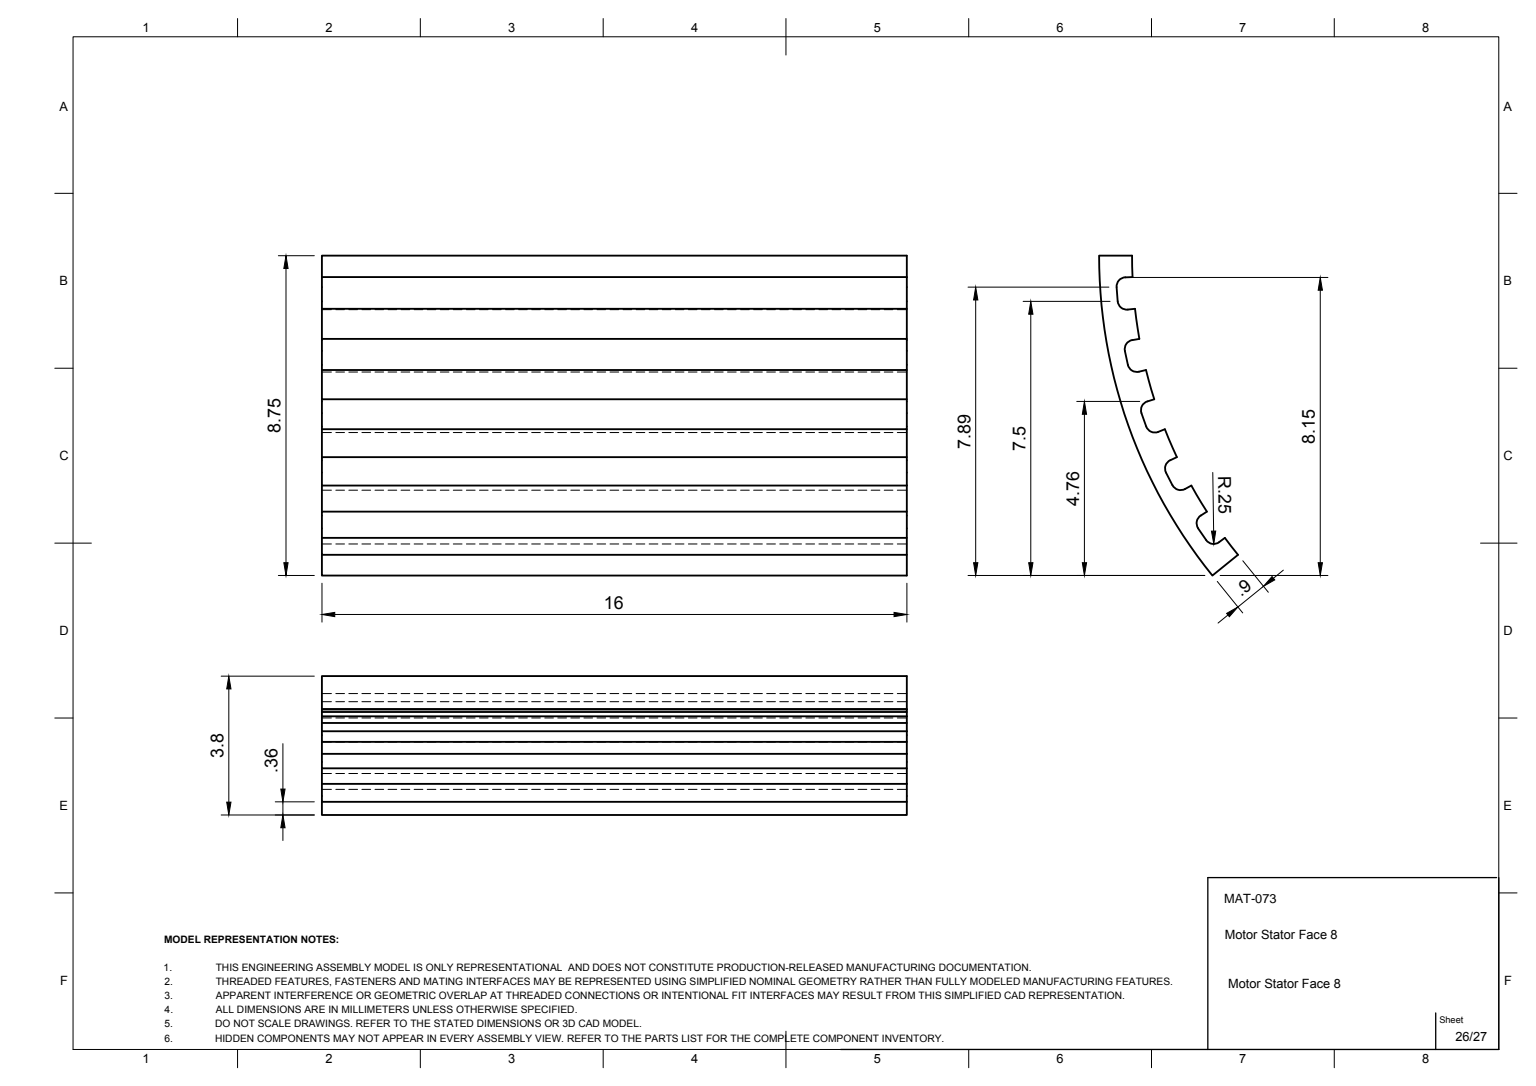
ISO-10303-21;
HEADER;
/* Generated by software containing ST-Developer
 * from STEP Tools, Inc. (www.steptools.com) 
 */

FILE_DESCRIPTION(
/* description */ ('CAx-IF Rec.Pracs.---Representation and Presentation of Product Manufa
cturing Information (PMI)---4.0---2014-10-13'),
/* implementation_level */ '2;1');

FILE_NAME(
/* name */ 'Motor Stator Face 8.step',
/* time_stamp */ '2026-10-24T18:52:33-07:00',
/* author */ (''),
/* organization */ (''),
/* preprocessor_version */ 'ST-DEVELOPER v20.2',
/* originating_system */ 'Autodesk Translation Framework v15.17.0.0',
/* authorisation */ '');

FILE_SCHEMA (('AP242_MANAGED_MODEL_BASED_3D_ENGINEERING_MIM_LF { 1 0 10303 442 2 1 4 }'));
ENDSEC;

DATA;
#10=MECHANICAL_DESIGN_GEOMETRIC_PRESENTATION_REPRESENTATION('',(#443),#34876);
#377=SHAPE_REPRESENTATION_RELATIONSHIP('SRR','None',#35014,#410);
#410=ADVANCED_BREP_SHAPE_REPRESENTATION('',(#476),#34872);
#443=STYLED_ITEM('',(#35163),#476);
#476=MANIFOLD_SOLID_BREP('Motor Stator Face 8',#19583);
#1049=PLANE('',#22059);
#1050=PLANE('',#22069);
#1051=PLANE('',#22079);
#1052=PLANE('',#22089);
#1053=PLANE('',#22099);
#1054=PLANE('',#22100);
#1055=PLANE('',#22101);
#1056=PLANE('',#22102);
#1057=PLANE('',#22103);
#1058=PLANE('',#22110);
#1059=PLANE('',#22120);
#1060=PLANE('',#22123);
#1061=PLANE('',#22126);
#1062=PLANE('',#22129);
#2589=LINE('',#34145,#4188);
#2590=LINE('',#34148,#4189);
#2591=LINE('',#34153,#4190);
#2592=LINE('',#34159,#4191);
#2593=LINE('',#34163,#4192);
#2594=LINE('',#34165,#4193);
#2595=LINE('',#34166,#4194);
#2596=LINE('',#34172,#4195);
#2597=LINE('',#34175,#4196);
#2598=LINE('',#34180,#4197);
#2599=LINE('',#34186,#4198);
#2600=LINE('',#34190,#4199);
#2601=LINE('',#34192,#4200);
#2602=LINE('',#34193,#4201);
#2603=LINE('',#34199,#4202);
#2604=LINE('',#34202,#4203);
#2605=LINE('',#34207,#4204);
#2606=LINE('',#34213,#4205);
#2607=LINE('',#34217,#4206);
#2608=LINE('',#34219,#4207);
#2609=LINE('',#34220,#4208);
#2610=LINE('',#34226,#4209);
#2611=LINE('',#34229,#4210);
#2612=LINE('',#34234,#4211);
#2613=LINE('',#34240,#4212);
#2614=LINE('',#34244,#4213);
#2615=LINE('',#34246,#4214);
#2616=LINE('',#34247,#4215);
#2617=LINE('',#34253,#4216);
#2618=LINE('',#34256,#4217);
#2619=LINE('',#34261,#4218);
#2620=LINE('',#34267,#4219);
#2621=LINE('',#34271,#4220);
#2622=LINE('',#34273,#4221);
#2623=LINE('',#34274,#4222);
#2624=LINE('',#34277,#4223);
#2625=LINE('',#34279,#4224);
#2626=LINE('',#34280,#4225);
#2627=LINE('',#34283,#4226);
#2628=LINE('',#34285,#4227);
#2629=LINE('',#34286,#4228);
#2630=LINE('',#34289,#4229);
#2631=LINE('',#34291,#4230);
#2632=LINE('',#34292,#4231);
#2633=LINE('',#34295,#4232);
#2634=LINE('',#34297,#4233);
#2635=LINE('',#34298,#4234);
#2636=LINE('',#34303,#4235);
#2637=LINE('',#34310,#4236);
#2638=LINE('',#34314,#4237);
#2639=LINE('',#34319,#4238);
#2640=LINE('',#34324,#4239);
#2641=LINE('',#34327,#4240);
#2642=LINE('',#34330,#4241);
#2643=LINE('',#34335,#4242);
#2644=LINE('',#34336,#4243);
#2645=LINE('',#34340,#4244);
#2646=LINE('',#34342,#4245);
#4188=VECTOR('',#27966,1.);
#4189=VECTOR('',#27969,1.);
#4190=VECTOR('',#27974,1.);
#4191=VECTOR('',#27981,1.);
#4192=VECTOR('',#27986,1.);
#4193=VECTOR('',#27987,1.);
#4194=VECTOR('',#27988,1.);
#4195=VECTOR('',#27993,1.);
#4196=VECTOR('',#27996,1.);
#4197=VECTOR('',#28001,1.);
#4198=VECTOR('',#28008,1.);
#4199=VECTOR('',#28013,0.999999999999999);
#4200=VECTOR('',#28014,1.);
#4201=VECTOR('',#28015,0.999999999999999);
#4202=VECTOR('',#28020,1.);
#4203=VECTOR('',#28023,1.);
#4204=VECTOR('',#28028,1.);
#4205=VECTOR('',#28035,1.);
#4206=VECTOR('',#28040,1.);
#4207=VECTOR('',#28041,1.);
#4208=VECTOR('',#28042,1.);
#4209=VECTOR('',#28047,1.);
#4210=VECTOR('',#28050,1.);
#4211=VECTOR('',#28055,1.);
#4212=VECTOR('',#28062,1.);
#4213=VECTOR('',#28067,1.);
#4214=VECTOR('',#28068,1.);
#4215=VECTOR('',#28069,1.);
#4216=VECTOR('',#28074,1.);
#4217=VECTOR('',#28077,1.);
#4218=VECTOR('',#28082,1.);
#4219=VECTOR('',#28089,1.);
#4220=VECTOR('',#28094,1.);
#4221=VECTOR('',#28095,1.);
#4222=VECTOR('',#28096,1.);
#4223=VECTOR('',#28099,1.);
#4224=VECTOR('',#28100,1.);
#4225=VECTOR('',#28101,1.);
#4226=VECTOR('',#28104,0.999999999999999);
#4227=VECTOR('',#28105,1.);
#4228=VECTOR('',#28106,0.999999999999999);
#4229=VECTOR('',#28109,1.);
#4230=VECTOR('',#28110,1.);
#4231=VECTOR('',#28111,1.);
#4232=VECTOR('',#28114,1.);
#4233=VECTOR('',#28115,1.);
#4234=VECTOR('',#28116,1.);
#4235=VECTOR('',#28121,1.);
#4236=VECTOR('',#28132,1.);
#4237=VECTOR('',#28135,1.);
#4238=VECTOR('',#28142,1.);
#4239=VECTOR('',#28149,1.);
#4240=VECTOR('',#28152,1.);
#4241=VECTOR('',#28157,1.);
#4242=VECTOR('',#28164,1.);
#4243=VECTOR('',#28165,1.);
#4244=VECTOR('',#28170,1.);
#4245=VECTOR('',#28173,1.);
#4766=CYLINDRICAL_SURFACE('',#22050,0.00025);
#4767=CYLINDRICAL_SURFACE('',#22053,0.01345);
#4768=CYLINDRICAL_SURFACE('',#22056,0.00025);
#4769=CYLINDRICAL_SURFACE('',#22060,0.00025);
#4770=CYLINDRICAL_SURFACE('',#22063,0.01345);
#4771=CYLINDRICAL_SURFACE('',#22066,0.00025);
#4772=CYLINDRICAL_SURFACE('',#22070,0.00025);
#4773=CYLINDRICAL_SURFACE('',#22073,0.01345);
#4774=CYLINDRICAL_SURFACE('',#22076,0.00025);
#4775=CYLINDRICAL_SURFACE('',#22080,0.00025);
#4776=CYLINDRICAL_SURFACE('',#22083,0.01345);
#4777=CYLINDRICAL_SURFACE('',#22086,0.00025);
#4778=CYLINDRICAL_SURFACE('',#22090,0.00025);
#4779=CYLINDRICAL_SURFACE('',#22093,0.01345);
#4780=CYLINDRICAL_SURFACE('',#22096,0.00025);
#4781=CYLINDRICAL_SURFACE('',#22104,0.013);
#4782=CYLINDRICAL_SURFACE('',#22107,0.013);
#4783=CYLINDRICAL_SURFACE('',#22116,0.013);
#4784=CYLINDRICAL_SURFACE('',#22118,0.013);
#4785=CYLINDRICAL_SURFACE('',#22121,0.013);
#4786=CYLINDRICAL_SURFACE('',#22124,0.0139);
#4787=CYLINDRICAL_SURFACE('',#22127,0.013);
#5757=FACE_OUTER_BOUND('',#6908,.T.);
#5758=FACE_OUTER_BOUND('',#6909,.T.);
#5759=FACE_OUTER_BOUND('',#6910,.T.);
#5760=FACE_OUTER_BOUND('',#6911,.T.);
#5761=FACE_OUTER_BOUND('',#6912,.T.);
#5762=FACE_OUTER_BOUND('',#6913,.T.);
#5763=FACE_OUTER_BOUND('',#6914,.T.);
#5764=FACE_OUTER_BOUND('',#6915,.T.);
#5765=FACE_OUTER_BOUND('',#6916,.T.);
#5766=FACE_OUTER_BOUND('',#6917,.T.);
#5767=FACE_OUTER_BOUND('',#6918,.T.);
#5768=FACE_OUTER_BOUND('',#6919,.T.);
#5769=FACE_OUTER_BOUND('',#6920,.T.);
#5770=FACE_OUTER_BOUND('',#6921,.T.);
#5771=FACE_OUTER_BOUND('',#6922,.T.);
#5772=FACE_OUTER_BOUND('',#6923,.T.);
#5773=FACE_OUTER_BOUND('',#6924,.T.);
#5774=FACE_OUTER_BOUND('',#6925,.T.);
#5775=FACE_OUTER_BOUND('',#6926,.T.);
#5776=FACE_OUTER_BOUND('',#6927,.T.);
#5777=FACE_OUTER_BOUND('',#6928,.T.);
#5778=FACE_OUTER_BOUND('',#6929,.T.);
#5779=FACE_OUTER_BOUND('',#6930,.T.);
#5780=FACE_OUTER_BOUND('',#6931,.T.);
#5781=FACE_OUTER_BOUND('',#6932,.T.);
#5782=FACE_OUTER_BOUND('',#6933,.T.);
#5783=FACE_OUTER_BOUND('',#6934,.T.);
#5784=FACE_OUTER_BOUND('',#6935,.T.);
#5785=FACE_OUTER_BOUND('',#6936,.T.);
#5786=FACE_OUTER_BOUND('',#6937,.T.);
#5787=FACE_OUTER_BOUND('',#6938,.T.);
#5788=FACE_OUTER_BOUND('',#6939,.T.);
#5789=FACE_OUTER_BOUND('',#6940,.T.);
#5790=FACE_OUTER_BOUND('',#6941,.T.);
#5791=FACE_OUTER_BOUND('',#6942,.T.);
#5792=FACE_OUTER_BOUND('',#6943,.T.);
#6908=EDGE_LOOP('',(#18070,#18071,#18072,#18073));
#6909=EDGE_LOOP('',(#18074,#18075,#18076,#18077));
#6910=EDGE_LOOP('',(#18078,#18079,#18080,#18081));
#6911=EDGE_LOOP('',(#18082,#18083,#18084,#18085));
#6912=EDGE_LOOP('',(#18086,#18087,#18088,#18089));
#6913=EDGE_LOOP('',(#18090,#18091,#18092,#18093));
#6914=EDGE_LOOP('',(#18094,#18095,#18096,#18097));
#6915=EDGE_LOOP('',(#18098,#18099,#18100,#18101));
#6916=EDGE_LOOP('',(#18102,#18103,#18104,#18105));
#6917=EDGE_LOOP('',(#18106,#18107,#18108,#18109));
#6918=EDGE_LOOP('',(#18110,#18111,#18112,#18113));
#6919=EDGE_LOOP('',(#18114,#18115,#18116,#18117));
#6920=EDGE_LOOP('',(#18118,#18119,#18120,#18121));
#6921=EDGE_LOOP('',(#18122,#18123,#18124,#18125));
#6922=EDGE_LOOP('',(#18126,#18127,#18128,#18129));
#6923=EDGE_LOOP('',(#18130,#18131,#18132,#18133));
#6924=EDGE_LOOP('',(#18134,#18135,#18136,#18137));
#6925=EDGE_LOOP('',(#18138,#18139,#18140,#18141));
#6926=EDGE_LOOP('',(#18142,#18143,#18144,#18145));
#6927=EDGE_LOOP('',(#18146,#18147,#18148,#18149));
#6928=EDGE_LOOP('',(#18150,#18151,#18152,#18153));
#6929=EDGE_LOOP('',(#18154,#18155,#18156,#18157));
#6930=EDGE_LOOP('',(#18158,#18159,#18160,#18161));
#6931=EDGE_LOOP('',(#18162,#18163,#18164,#18165));
#6932=EDGE_LOOP('',(#18166,#18167,#18168,#18169));
#6933=EDGE_LOOP('',(#18170,#18171,#18172,#18173));
#6934=EDGE_LOOP('',(#18174,#18175,#18176,#18177,#18178,#18179,#18180,#18181,
#18182,#18183,#18184,#18185,#18186,#18187,#18188,#18189,#18190,#18191,#18192,
#18193,#18194,#18195,#18196,#18197,#18198,#18199,#18200,#18201,#18202,#18203,
#18204,#18205,#18206,#18207));
#6935=EDGE_LOOP('',(#18208,#18209,#18210,#18211));
#6936=EDGE_LOOP('',(#18212,#18213,#18214,#18215));
#6937=EDGE_LOOP('',(#18216,#18217,#18218,#18219));
#6938=EDGE_LOOP('',(#18220,#18221,#18222,#18223));
#6939=EDGE_LOOP('',(#18224,#18225,#18226,#18227));
#6940=EDGE_LOOP('',(#18228,#18229,#18230,#18231));
#6941=EDGE_LOOP('',(#18232,#18233,#18234,#18235));
#6942=EDGE_LOOP('',(#18236,#18237,#18238,#18239));
#6943=EDGE_LOOP('',(#18240,#18241,#18242,#18243,#18244,#18245,#18246,#18247,
#18248,#18249,#18250,#18251,#18252,#18253,#18254,#18255,#18256,#18257,#18258,
#18259,#18260,#18261,#18262,#18263,#18264,#18265,#18266,#18267,#18268,#18269,
#18270,#18271,#18272,#18273));
#7985=CIRCLE('',#22051,0.000250000000012414);
#7986=CIRCLE('',#22052,0.000250000000012414);
#7987=CIRCLE('',#22054,0.0134500000000135);
#7988=CIRCLE('',#22055,0.0134500000000135);
#7989=CIRCLE('',#22057,0.000250000000012074);
#7990=CIRCLE('',#22058,0.000250000000012074);
#7991=CIRCLE('',#22061,0.000250000000011423);
#7992=CIRCLE('',#22062,0.000250000000011423);
#7993=CIRCLE('',#22064,0.0134500000000139);
#7994=CIRCLE('',#22065,0.0134500000000139);
#7995=CIRCLE('',#22067,0.00025000000001101);
#7996=CIRCLE('',#22068,0.00025000000001101);
#7997=CIRCLE('',#22071,0.000250000000010237);
#7998=CIRCLE('',#22072,0.000250000000010237);
#7999=CIRCLE('',#22074,0.0134500000000141);
#8000=CIRCLE('',#22075,0.0134500000000141);
#8001=CIRCLE('',#22077,0.000250000000010237);
#8002=CIRCLE('',#22078,0.000250000000010237);
#8003=CIRCLE('',#22081,0.00025000000001101);
#8004=CIRCLE('',#22082,0.00025000000001101);
#8005=CIRCLE('',#22084,0.0134500000000141);
#8006=CIRCLE('',#22085,0.0134500000000141);
#8007=CIRCLE('',#22087,0.000250000000011423);
#8008=CIRCLE('',#22088,0.000250000000011423);
#8009=CIRCLE('',#22091,0.000250000000012074);
#8010=CIRCLE('',#22092,0.000250000000012074);
#8011=CIRCLE('',#22094,0.0134500000000138);
#8012=CIRCLE('',#22095,0.0134500000000138);
#8013=CIRCLE('',#22097,0.000250000000012414);
#8014=CIRCLE('',#22098,0.000250000000012414);
#8015=CIRCLE('',#22105,0.0130000000000133);
#8016=CIRCLE('',#22106,0.0130000000000133);
#8017=CIRCLE('',#22108,0.0130000000000133);
#8018=CIRCLE('',#22109,0.0130000000000133);
#8019=CIRCLE('',#22111,0.0139000000000133);
#8020=CIRCLE('',#22112,0.0130000000000133);
#8021=CIRCLE('',#22113,0.0130000000000133);
#8022=CIRCLE('',#22114,0.0130000000000133);
#8023=CIRCLE('',#22115,0.0130000000000133);
#8024=CIRCLE('',#22117,0.0130000000000133);
#8025=CIRCLE('',#22119,0.0130000000000133);
#8026=CIRCLE('',#22122,0.0130000000000133);
#8027=CIRCLE('',#22125,0.0139000000000133);
#8028=CIRCLE('',#22128,0.0130000000000133);
#9819=VERTEX_POINT('',#34141);
#9820=VERTEX_POINT('',#34142);
#9821=VERTEX_POINT('',#34144);
#9822=VERTEX_POINT('',#34146);
#9823=VERTEX_POINT('',#34150);
#9824=VERTEX_POINT('',#34152);
#9825=VERTEX_POINT('',#34156);
#9826=VERTEX_POINT('',#34158);
#9827=VERTEX_POINT('',#34162);
#9828=VERTEX_POINT('',#34164);
#9829=VERTEX_POINT('',#34168);
#9830=VERTEX_POINT('',#34169);
#9831=VERTEX_POINT('',#34171);
#9832=VERTEX_POINT('',#34173);
#9833=VERTEX_POINT('',#34177);
#9834=VERTEX_POINT('',#34179);
#9835=VERTEX_POINT('',#34183);
#9836=VERTEX_POINT('',#34185);
#9837=VERTEX_POINT('',#34189);
#9838=VERTEX_POINT('',#34191);
#9839=VERTEX_POINT('',#34195);
#9840=VERTEX_POINT('',#34196);
#9841=VERTEX_POINT('',#34198);
#9842=VERTEX_POINT('',#34200);
#9843=VERTEX_POINT('',#34204);
#9844=VERTEX_POINT('',#34206);
#9845=VERTEX_POINT('',#34210);
#9846=VERTEX_POINT('',#34212);
#9847=VERTEX_POINT('',#34216);
#9848=VERTEX_POINT('',#34218);
#9849=VERTEX_POINT('',#34222);
#9850=VERTEX_POINT('',#34223);
#9851=VERTEX_POINT('',#34225);
#9852=VERTEX_POINT('',#34227);
#9853=VERTEX_POINT('',#34231);
#9854=VERTEX_POINT('',#34233);
#9855=VERTEX_POINT('',#34237);
#9856=VERTEX_POINT('',#34239);
#9857=VERTEX_POINT('',#34243);
#9858=VERTEX_POINT('',#34245);
#9859=VERTEX_POINT('',#34249);
#9860=VERTEX_POINT('',#34250);
#9861=VERTEX_POINT('',#34252);
#9862=VERTEX_POINT('',#34254);
#9863=VERTEX_POINT('',#34258);
#9864=VERTEX_POINT('',#34260);
#9865=VERTEX_POINT('',#34264);
#9866=VERTEX_POINT('',#34266);
#9867=VERTEX_POINT('',#34270);
#9868=VERTEX_POINT('',#34272);
#9869=VERTEX_POINT('',#34276);
#9870=VERTEX_POINT('',#34278);
#9871=VERTEX_POINT('',#34282);
#9872=VERTEX_POINT('',#34284);
#9873=VERTEX_POINT('',#34288);
#9874=VERTEX_POINT('',#34290);
#9875=VERTEX_POINT('',#34294);
#9876=VERTEX_POINT('',#34296);
#9877=VERTEX_POINT('',#34300);
#9878=VERTEX_POINT('',#34302);
#9879=VERTEX_POINT('',#34309);
#9880=VERTEX_POINT('',#34311);
#9881=VERTEX_POINT('',#34313);
#9882=VERTEX_POINT('',#34317);
#9883=VERTEX_POINT('',#34322);
#9884=VERTEX_POINT('',#34326);
#9885=VERTEX_POINT('',#34334);
#9886=VERTEX_POINT('',#34338);
#12593=EDGE_CURVE('',#9819,#9820,#7985,.T.);
#12594=EDGE_CURVE('',#9820,#9821,#2589,.T.);
#12595=EDGE_CURVE('',#9821,#9822,#7986,.T.);
#12596=EDGE_CURVE('',#9822,#9819,#2590,.T.);
#12597=EDGE_CURVE('',#9823,#9820,#7987,.T.);
#12598=EDGE_CURVE('',#9824,#9823,#2591,.T.);
#12599=EDGE_CURVE('',#9821,#9824,#7988,.T.);
#12600=EDGE_CURVE('',#9823,#9825,#7989,.T.);
#12601=EDGE_CURVE('',#9825,#9826,#2592,.T.);
#12602=EDGE_CURVE('',#9826,#9824,#7990,.T.);
#12603=EDGE_CURVE('',#9827,#9825,#2593,.T.);
#12604=EDGE_CURVE('',#9828,#9827,#2594,.T.);
#12605=EDGE_CURVE('',#9826,#9828,#2595,.T.);
#12606=EDGE_CURVE('',#9829,#9830,#7991,.T.);
#12607=EDGE_CURVE('',#9830,#9831,#2596,.T.);
#12608=EDGE_CURVE('',#9831,#9832,#7992,.T.);
#12609=EDGE_CURVE('',#9832,#9829,#2597,.T.);
#12610=EDGE_CURVE('',#9833,#9830,#7993,.T.);
#12611=EDGE_CURVE('',#9834,#9833,#2598,.T.);
#12612=EDGE_CURVE('',#9831,#9834,#7994,.T.);
#12613=EDGE_CURVE('',#9833,#9835,#7995,.T.);
#12614=EDGE_CURVE('',#9835,#9836,#2599,.T.);
#12615=EDGE_CURVE('',#9836,#9834,#7996,.T.);
#12616=EDGE_CURVE('',#9837,#9835,#2600,.T.);
#12617=EDGE_CURVE('',#9838,#9837,#2601,.T.);
#12618=EDGE_CURVE('',#9836,#9838,#2602,.T.);
#12619=EDGE_CURVE('',#9839,#9840,#7997,.T.);
#12620=EDGE_CURVE('',#9840,#9841,#2603,.T.);
#12621=EDGE_CURVE('',#9841,#9842,#7998,.T.);
#12622=EDGE_CURVE('',#9842,#9839,#2604,.T.);
#12623=EDGE_CURVE('',#9843,#9840,#7999,.T.);
#12624=EDGE_CURVE('',#9844,#9843,#2605,.T.);
#12625=EDGE_CURVE('',#9841,#9844,#8000,.T.);
#12626=EDGE_CURVE('',#9843,#9845,#8001,.T.);
#12627=EDGE_CURVE('',#9845,#9846,#2606,.T.);
#12628=EDGE_CURVE('',#9846,#9844,#8002,.T.);
#12629=EDGE_CURVE('',#9847,#9845,#2607,.T.);
#12630=EDGE_CURVE('',#9848,#9847,#2608,.T.);
#12631=EDGE_CURVE('',#9846,#9848,#2609,.T.);
#12632=EDGE_CURVE('',#9849,#9850,#8003,.T.);
#12633=EDGE_CURVE('',#9850,#9851,#2610,.T.);
#12634=EDGE_CURVE('',#9851,#9852,#8004,.T.);
#12635=EDGE_CURVE('',#9852,#9849,#2611,.T.);
#12636=EDGE_CURVE('',#9853,#9850,#8005,.T.);
#12637=EDGE_CURVE('',#9854,#9853,#2612,.T.);
#12638=EDGE_CURVE('',#9851,#9854,#8006,.T.);
#12639=EDGE_CURVE('',#9853,#9855,#8007,.T.);
#12640=EDGE_CURVE('',#9855,#9856,#2613,.T.);
#12641=EDGE_CURVE('',#9856,#9854,#8008,.T.);
#12642=EDGE_CURVE('',#9857,#9855,#2614,.T.);
#12643=EDGE_CURVE('',#9858,#9857,#2615,.T.);
#12644=EDGE_CURVE('',#9856,#9858,#2616,.T.);
#12645=EDGE_CURVE('',#9859,#9860,#8009,.T.);
#12646=EDGE_CURVE('',#9860,#9861,#2617,.T.);
#12647=EDGE_CURVE('',#9861,#9862,#8010,.T.);
#12648=EDGE_CURVE('',#9862,#9859,#2618,.T.);
#12649=EDGE_CURVE('',#9863,#9860,#8011,.T.);
#12650=EDGE_CURVE('',#9864,#9863,#2619,.T.);
#12651=EDGE_CURVE('',#9861,#9864,#8012,.T.);
#12652=EDGE_CURVE('',#9863,#9865,#8013,.T.);
#12653=EDGE_CURVE('',#9865,#9866,#2620,.T.);
#12654=EDGE_CURVE('',#9866,#9864,#8014,.T.);
#12655=EDGE_CURVE('',#9867,#9865,#2621,.T.);
#12656=EDGE_CURVE('',#9868,#9867,#2622,.T.);
#12657=EDGE_CURVE('',#9866,#9868,#2623,.T.);
#12658=EDGE_CURVE('',#9869,#9862,#2624,.T.);
#12659=EDGE_CURVE('',#9870,#9869,#2625,.T.);
#12660=EDGE_CURVE('',#9859,#9870,#2626,.T.);
#12661=EDGE_CURVE('',#9871,#9852,#2627,.T.);
#12662=EDGE_CURVE('',#9872,#9871,#2628,.T.);
#12663=EDGE_CURVE('',#9849,#9872,#2629,.T.);
#12664=EDGE_CURVE('',#9873,#9832,#2630,.T.);
#12665=EDGE_CURVE('',#9874,#9873,#2631,.T.);
#12666=EDGE_CURVE('',#9829,#9874,#2632,.T.);
#12667=EDGE_CURVE('',#9875,#9822,#2633,.T.);
#12668=EDGE_CURVE('',#9876,#9875,#2634,.T.);
#12669=EDGE_CURVE('',#9819,#9876,#2635,.T.);
#12670=EDGE_CURVE('',#9877,#9867,#8015,.T.);
#12671=EDGE_CURVE('',#9877,#9878,#2636,.T.);
#12672=EDGE_CURVE('',#9868,#9878,#8016,.T.);
#12673=EDGE_CURVE('',#9848,#9871,#8017,.T.);
#12674=EDGE_CURVE('',#9872,#9847,#8018,.T.);
#12675=EDGE_CURVE('',#9878,#9879,#2637,.T.);
#12676=EDGE_CURVE('',#9879,#9880,#8019,.T.);
#12677=EDGE_CURVE('',#9880,#9881,#2638,.T.);
#12678=EDGE_CURVE('',#9881,#9875,#8020,.T.);
#12679=EDGE_CURVE('',#9828,#9873,#8021,.T.);
#12680=EDGE_CURVE('',#9838,#9882,#8022,.T.);
#12681=EDGE_CURVE('',#9882,#9842,#2639,.T.);
#12682=EDGE_CURVE('',#9858,#9869,#8023,.T.);
#12683=EDGE_CURVE('',#9883,#9837,#8024,.T.);
#12684=EDGE_CURVE('',#9883,#9882,#2640,.T.);
#12685=EDGE_CURVE('',#9881,#9884,#2641,.T.);
#12686=EDGE_CURVE('',#9876,#9884,#8025,.T.);
#12687=EDGE_CURVE('',#9839,#9883,#2642,.T.);
#12688=EDGE_CURVE('',#9870,#9857,#8026,.T.);
#12689=EDGE_CURVE('',#9885,#9877,#2643,.T.);
#12690=EDGE_CURVE('',#9879,#9885,#2644,.T.);
#12691=EDGE_CURVE('',#9886,#9885,#8027,.T.);
#12692=EDGE_CURVE('',#9880,#9886,#2645,.T.);
#12693=EDGE_CURVE('',#9884,#9886,#2646,.T.);
#12694=EDGE_CURVE('',#9874,#9827,#8028,.T.);
#18070=ORIENTED_EDGE('',*,*,#12593,.T.);
#18071=ORIENTED_EDGE('',*,*,#12594,.T.);
#18072=ORIENTED_EDGE('',*,*,#12595,.T.);
#18073=ORIENTED_EDGE('',*,*,#12596,.T.);
#18074=ORIENTED_EDGE('',*,*,#12594,.F.);
#18075=ORIENTED_EDGE('',*,*,#12597,.F.);
#18076=ORIENTED_EDGE('',*,*,#12598,.F.);
#18077=ORIENTED_EDGE('',*,*,#12599,.F.);
#18078=ORIENTED_EDGE('',*,*,#12600,.T.);
#18079=ORIENTED_EDGE('',*,*,#12601,.T.);
#18080=ORIENTED_EDGE('',*,*,#12602,.T.);
#18081=ORIENTED_EDGE('',*,*,#12598,.T.);
#18082=ORIENTED_EDGE('',*,*,#12601,.F.);
#18083=ORIENTED_EDGE('',*,*,#12603,.F.);
#18084=ORIENTED_EDGE('',*,*,#12604,.F.);
#18085=ORIENTED_EDGE('',*,*,#12605,.F.);
#18086=ORIENTED_EDGE('',*,*,#12606,.T.);
#18087=ORIENTED_EDGE('',*,*,#12607,.T.);
#18088=ORIENTED_EDGE('',*,*,#12608,.T.);
#18089=ORIENTED_EDGE('',*,*,#12609,.T.);
#18090=ORIENTED_EDGE('',*,*,#12607,.F.);
#18091=ORIENTED_EDGE('',*,*,#12610,.F.);
#18092=ORIENTED_EDGE('',*,*,#12611,.F.);
#18093=ORIENTED_EDGE('',*,*,#12612,.F.);
#18094=ORIENTED_EDGE('',*,*,#12613,.T.);
#18095=ORIENTED_EDGE('',*,*,#12614,.T.);
#18096=ORIENTED_EDGE('',*,*,#12615,.T.);
#18097=ORIENTED_EDGE('',*,*,#12611,.T.);
#18098=ORIENTED_EDGE('',*,*,#12614,.F.);
#18099=ORIENTED_EDGE('',*,*,#12616,.F.);
#18100=ORIENTED_EDGE('',*,*,#12617,.F.);
#18101=ORIENTED_EDGE('',*,*,#12618,.F.);
#18102=ORIENTED_EDGE('',*,*,#12619,.T.);
#18103=ORIENTED_EDGE('',*,*,#12620,.T.);
#18104=ORIENTED_EDGE('',*,*,#12621,.T.);
#18105=ORIENTED_EDGE('',*,*,#12622,.T.);
#18106=ORIENTED_EDGE('',*,*,#12620,.F.);
#18107=ORIENTED_EDGE('',*,*,#12623,.F.);
#18108=ORIENTED_EDGE('',*,*,#12624,.F.);
#18109=ORIENTED_EDGE('',*,*,#12625,.F.);
#18110=ORIENTED_EDGE('',*,*,#12626,.T.);
#18111=ORIENTED_EDGE('',*,*,#12627,.T.);
#18112=ORIENTED_EDGE('',*,*,#12628,.T.);
#18113=ORIENTED_EDGE('',*,*,#12624,.T.);
#18114=ORIENTED_EDGE('',*,*,#12627,.F.);
#18115=ORIENTED_EDGE('',*,*,#12629,.F.);
#18116=ORIENTED_EDGE('',*,*,#12630,.F.);
#18117=ORIENTED_EDGE('',*,*,#12631,.F.);
#18118=ORIENTED_EDGE('',*,*,#12632,.T.);
#18119=ORIENTED_EDGE('',*,*,#12633,.T.);
#18120=ORIENTED_EDGE('',*,*,#12634,.T.);
#18121=ORIENTED_EDGE('',*,*,#12635,.T.);
#18122=ORIENTED_EDGE('',*,*,#12633,.F.);
#18123=ORIENTED_EDGE('',*,*,#12636,.F.);
#18124=ORIENTED_EDGE('',*,*,#12637,.F.);
#18125=ORIENTED_EDGE('',*,*,#12638,.F.);
#18126=ORIENTED_EDGE('',*,*,#12639,.T.);
#18127=ORIENTED_EDGE('',*,*,#12640,.T.);
#18128=ORIENTED_EDGE('',*,*,#12641,.T.);
#18129=ORIENTED_EDGE('',*,*,#12637,.T.);
#18130=ORIENTED_EDGE('',*,*,#12640,.F.);
#18131=ORIENTED_EDGE('',*,*,#12642,.F.);
#18132=ORIENTED_EDGE('',*,*,#12643,.F.);
#18133=ORIENTED_EDGE('',*,*,#12644,.F.);
#18134=ORIENTED_EDGE('',*,*,#12645,.T.);
#18135=ORIENTED_EDGE('',*,*,#12646,.T.);
#18136=ORIENTED_EDGE('',*,*,#12647,.T.);
#18137=ORIENTED_EDGE('',*,*,#12648,.T.);
#18138=ORIENTED_EDGE('',*,*,#12646,.F.);
#18139=ORIENTED_EDGE('',*,*,#12649,.F.);
#18140=ORIENTED_EDGE('',*,*,#12650,.F.);
#18141=ORIENTED_EDGE('',*,*,#12651,.F.);
#18142=ORIENTED_EDGE('',*,*,#12652,.T.);
#18143=ORIENTED_EDGE('',*,*,#12653,.T.);
#18144=ORIENTED_EDGE('',*,*,#12654,.T.);
#18145=ORIENTED_EDGE('',*,*,#12650,.T.);
#18146=ORIENTED_EDGE('',*,*,#12653,.F.);
#18147=ORIENTED_EDGE('',*,*,#12655,.F.);
#18148=ORIENTED_EDGE('',*,*,#12656,.F.);
#18149=ORIENTED_EDGE('',*,*,#12657,.F.);
#18150=ORIENTED_EDGE('',*,*,#12648,.F.);
#18151=ORIENTED_EDGE('',*,*,#12658,.F.);
#18152=ORIENTED_EDGE('',*,*,#12659,.F.);
#18153=ORIENTED_EDGE('',*,*,#12660,.F.);
#18154=ORIENTED_EDGE('',*,*,#12635,.F.);
#18155=ORIENTED_EDGE('',*,*,#12661,.F.);
#18156=ORIENTED_EDGE('',*,*,#12662,.F.);
#18157=ORIENTED_EDGE('',*,*,#12663,.F.);
#18158=ORIENTED_EDGE('',*,*,#12609,.F.);
#18159=ORIENTED_EDGE('',*,*,#12664,.F.);
#18160=ORIENTED_EDGE('',*,*,#12665,.F.);
#18161=ORIENTED_EDGE('',*,*,#12666,.F.);
#18162=ORIENTED_EDGE('',*,*,#12596,.F.);
#18163=ORIENTED_EDGE('',*,*,#12667,.F.);
#18164=ORIENTED_EDGE('',*,*,#12668,.F.);
#18165=ORIENTED_EDGE('',*,*,#12669,.F.);
#18166=ORIENTED_EDGE('',*,*,#12656,.T.);
#18167=ORIENTED_EDGE('',*,*,#12670,.F.);
#18168=ORIENTED_EDGE('',*,*,#12671,.T.);
#18169=ORIENTED_EDGE('',*,*,#12672,.F.);
#18170=ORIENTED_EDGE('',*,*,#12662,.T.);
#18171=ORIENTED_EDGE('',*,*,#12673,.F.);
#18172=ORIENTED_EDGE('',*,*,#12630,.T.);
#18173=ORIENTED_EDGE('',*,*,#12674,.F.);
#18174=ORIENTED_EDGE('',*,*,#12658,.T.);
#18175=ORIENTED_EDGE('',*,*,#12647,.F.);
#18176=ORIENTED_EDGE('',*,*,#12651,.T.);
#18177=ORIENTED_EDGE('',*,*,#12654,.F.);
#18178=ORIENTED_EDGE('',*,*,#12657,.T.);
#18179=ORIENTED_EDGE('',*,*,#12672,.T.);
#18180=ORIENTED_EDGE('',*,*,#12675,.T.);
#18181=ORIENTED_EDGE('',*,*,#12676,.T.);
#18182=ORIENTED_EDGE('',*,*,#12677,.T.);
#18183=ORIENTED_EDGE('',*,*,#12678,.T.);
#18184=ORIENTED_EDGE('',*,*,#12667,.T.);
#18185=ORIENTED_EDGE('',*,*,#12595,.F.);
#18186=ORIENTED_EDGE('',*,*,#12599,.T.);
#18187=ORIENTED_EDGE('',*,*,#12602,.F.);
#18188=ORIENTED_EDGE('',*,*,#12605,.T.);
#18189=ORIENTED_EDGE('',*,*,#12679,.T.);
#18190=ORIENTED_EDGE('',*,*,#12664,.T.);
#18191=ORIENTED_EDGE('',*,*,#12608,.F.);
#18192=ORIENTED_EDGE('',*,*,#12612,.T.);
#18193=ORIENTED_EDGE('',*,*,#12615,.F.);
#18194=ORIENTED_EDGE('',*,*,#12618,.T.);
#18195=ORIENTED_EDGE('',*,*,#12680,.T.);
#18196=ORIENTED_EDGE('',*,*,#12681,.T.);
#18197=ORIENTED_EDGE('',*,*,#12621,.F.);
#18198=ORIENTED_EDGE('',*,*,#12625,.T.);
#18199=ORIENTED_EDGE('',*,*,#12628,.F.);
#18200=ORIENTED_EDGE('',*,*,#12631,.T.);
#18201=ORIENTED_EDGE('',*,*,#12673,.T.);
#18202=ORIENTED_EDGE('',*,*,#12661,.T.);
#18203=ORIENTED_EDGE('',*,*,#12634,.F.);
#18204=ORIENTED_EDGE('',*,*,#12638,.T.);
#18205=ORIENTED_EDGE('',*,*,#12641,.F.);
#18206=ORIENTED_EDGE('',*,*,#12644,.T.);
#18207=ORIENTED_EDGE('',*,*,#12682,.T.);
#18208=ORIENTED_EDGE('',*,*,#12617,.T.);
#18209=ORIENTED_EDGE('',*,*,#12683,.F.);
#18210=ORIENTED_EDGE('',*,*,#12684,.T.);
#18211=ORIENTED_EDGE('',*,*,#12680,.F.);
#18212=ORIENTED_EDGE('',*,*,#12668,.T.);
#18213=ORIENTED_EDGE('',*,*,#12678,.F.);
#18214=ORIENTED_EDGE('',*,*,#12685,.T.);
#18215=ORIENTED_EDGE('',*,*,#12686,.F.);
#18216=ORIENTED_EDGE('',*,*,#12622,.F.);
#18217=ORIENTED_EDGE('',*,*,#12681,.F.);
#18218=ORIENTED_EDGE('',*,*,#12684,.F.);
#18219=ORIENTED_EDGE('',*,*,#12687,.F.);
#18220=ORIENTED_EDGE('',*,*,#12659,.T.);
#18221=ORIENTED_EDGE('',*,*,#12682,.F.);
#18222=ORIENTED_EDGE('',*,*,#12643,.T.);
#18223=ORIENTED_EDGE('',*,*,#12688,.F.);
#18224=ORIENTED_EDGE('',*,*,#12671,.F.);
#18225=ORIENTED_EDGE('',*,*,#12689,.F.);
#18226=ORIENTED_EDGE('',*,*,#12690,.F.);
#18227=ORIENTED_EDGE('',*,*,#12675,.F.);
#18228=ORIENTED_EDGE('',*,*,#12690,.T.);
#18229=ORIENTED_EDGE('',*,*,#12691,.F.);
#18230=ORIENTED_EDGE('',*,*,#12692,.F.);
#18231=ORIENTED_EDGE('',*,*,#12676,.F.);
#18232=ORIENTED_EDGE('',*,*,#12692,.T.);
#18233=ORIENTED_EDGE('',*,*,#12693,.F.);
#18234=ORIENTED_EDGE('',*,*,#12685,.F.);
#18235=ORIENTED_EDGE('',*,*,#12677,.F.);
#18236=ORIENTED_EDGE('',*,*,#12665,.T.);
#18237=ORIENTED_EDGE('',*,*,#12679,.F.);
#18238=ORIENTED_EDGE('',*,*,#12604,.T.);
#18239=ORIENTED_EDGE('',*,*,#12694,.F.);
#18240=ORIENTED_EDGE('',*,*,#12660,.T.);
#18241=ORIENTED_EDGE('',*,*,#12688,.T.);
#18242=ORIENTED_EDGE('',*,*,#12642,.T.);
#18243=ORIENTED_EDGE('',*,*,#12639,.F.);
#18244=ORIENTED_EDGE('',*,*,#12636,.T.);
#18245=ORIENTED_EDGE('',*,*,#12632,.F.);
#18246=ORIENTED_EDGE('',*,*,#12663,.T.);
#18247=ORIENTED_EDGE('',*,*,#12674,.T.);
#18248=ORIENTED_EDGE('',*,*,#12629,.T.);
#18249=ORIENTED_EDGE('',*,*,#12626,.F.);
#18250=ORIENTED_EDGE('',*,*,#12623,.T.);
#18251=ORIENTED_EDGE('',*,*,#12619,.F.);
#18252=ORIENTED_EDGE('',*,*,#12687,.T.);
#18253=ORIENTED_EDGE('',*,*,#12683,.T.);
#18254=ORIENTED_EDGE('',*,*,#12616,.T.);
#18255=ORIENTED_EDGE('',*,*,#12613,.F.);
#18256=ORIENTED_EDGE('',*,*,#12610,.T.);
#18257=ORIENTED_EDGE('',*,*,#12606,.F.);
#18258=ORIENTED_EDGE('',*,*,#12666,.T.);
#18259=ORIENTED_EDGE('',*,*,#12694,.T.);
#18260=ORIENTED_EDGE('',*,*,#12603,.T.);
#18261=ORIENTED_EDGE('',*,*,#12600,.F.);
#18262=ORIENTED_EDGE('',*,*,#12597,.T.);
#18263=ORIENTED_EDGE('',*,*,#12593,.F.);
#18264=ORIENTED_EDGE('',*,*,#12669,.T.);
#18265=ORIENTED_EDGE('',*,*,#12686,.T.);
#18266=ORIENTED_EDGE('',*,*,#12693,.T.);
#18267=ORIENTED_EDGE('',*,*,#12691,.T.);
#18268=ORIENTED_EDGE('',*,*,#12689,.T.);
#18269=ORIENTED_EDGE('',*,*,#12670,.T.);
#18270=ORIENTED_EDGE('',*,*,#12655,.T.);
#18271=ORIENTED_EDGE('',*,*,#12652,.F.);
#18272=ORIENTED_EDGE('',*,*,#12649,.T.);
#18273=ORIENTED_EDGE('',*,*,#12645,.F.);
#19473=ADVANCED_FACE('',(#5757),#4766,.F.);
#19474=ADVANCED_FACE('',(#5758),#4767,.F.);
#19475=ADVANCED_FACE('',(#5759),#4768,.F.);
#19476=ADVANCED_FACE('',(#5760),#1049,.F.);
#19477=ADVANCED_FACE('',(#5761),#4769,.F.);
#19478=ADVANCED_FACE('',(#5762),#4770,.F.);
#19479=ADVANCED_FACE('',(#5763),#4771,.F.);
#19480=ADVANCED_FACE('',(#5764),#1050,.F.);
#19481=ADVANCED_FACE('',(#5765),#4772,.F.);
#19482=ADVANCED_FACE('',(#5766),#4773,.F.);
#19483=ADVANCED_FACE('',(#5767),#4774,.F.);
#19484=ADVANCED_FACE('',(#5768),#1051,.F.);
#19485=ADVANCED_FACE('',(#5769),#4775,.F.);
#19486=ADVANCED_FACE('',(#5770),#4776,.F.);
#19487=ADVANCED_FACE('',(#5771),#4777,.F.);
#19488=ADVANCED_FACE('',(#5772),#1052,.F.);
#19489=ADVANCED_FACE('',(#5773),#4778,.F.);
#19490=ADVANCED_FACE('',(#5774),#4779,.F.);
#19491=ADVANCED_FACE('',(#5775),#4780,.F.);
#19492=ADVANCED_FACE('',(#5776),#1053,.F.);
#19493=ADVANCED_FACE('',(#5777),#1054,.F.);
#19494=ADVANCED_FACE('',(#5778),#1055,.F.);
#19495=ADVANCED_FACE('',(#5779),#1056,.F.);
#19496=ADVANCED_FACE('',(#5780),#1057,.F.);
#19497=ADVANCED_FACE('',(#5781),#4781,.F.);
#19498=ADVANCED_FACE('',(#5782),#4782,.F.);
#19499=ADVANCED_FACE('',(#5783),#1058,.F.);
#19500=ADVANCED_FACE('',(#5784),#4783,.F.);
#19501=ADVANCED_FACE('',(#5785),#4784,.F.);
#19502=ADVANCED_FACE('',(#5786),#1059,.F.);
#19503=ADVANCED_FACE('',(#5787),#4785,.F.);
#19504=ADVANCED_FACE('',(#5788),#1060,.T.);
#19505=ADVANCED_FACE('',(#5789),#4786,.T.);
#19506=ADVANCED_FACE('',(#5790),#1061,.T.);
#19507=ADVANCED_FACE('',(#5791),#4787,.F.);
#19508=ADVANCED_FACE('',(#5792),#1062,.T.);
#19583=CLOSED_SHELL('',(#19473,#19474,#19475,#19476,#19477,#19478,#19479,
#19480,#19481,#19482,#19483,#19484,#19485,#19486,#19487,#19488,#19489,#19490,
#19491,#19492,#19493,#19494,#19495,#19496,#19497,#19498,#19499,#19500,#19501,
#19502,#19503,#19504,#19505,#19506,#19507,#19508));
#22049=AXIS2_PLACEMENT_3D('',#34139,#27960,#27961);
#22050=AXIS2_PLACEMENT_3D('',#34140,#27962,#27963);
#22051=AXIS2_PLACEMENT_3D('',#34143,#27964,#27965);
#22052=AXIS2_PLACEMENT_3D('',#34147,#27967,#27968);
#22053=AXIS2_PLACEMENT_3D('',#34149,#27970,#27971);
#22054=AXIS2_PLACEMENT_3D('',#34151,#27972,#27973);
#22055=AXIS2_PLACEMENT_3D('',#34154,#27975,#27976);
#22056=AXIS2_PLACEMENT_3D('',#34155,#27977,#27978);
#22057=AXIS2_PLACEMENT_3D('',#34157,#27979,#27980);
#22058=AXIS2_PLACEMENT_3D('',#34160,#27982,#27983);
#22059=AXIS2_PLACEMENT_3D('',#34161,#27984,#27985);
#22060=AXIS2_PLACEMENT_3D('',#34167,#27989,#27990);
#22061=AXIS2_PLACEMENT_3D('',#34170,#27991,#27992);
#22062=AXIS2_PLACEMENT_3D('',#34174,#27994,#27995);
#22063=AXIS2_PLACEMENT_3D('',#34176,#27997,#27998);
#22064=AXIS2_PLACEMENT_3D('',#34178,#27999,#28000);
#22065=AXIS2_PLACEMENT_3D('',#34181,#28002,#28003);
#22066=AXIS2_PLACEMENT_3D('',#34182,#28004,#28005);
#22067=AXIS2_PLACEMENT_3D('',#34184,#28006,#28007);
#22068=AXIS2_PLACEMENT_3D('',#34187,#28009,#28010);
#22069=AXIS2_PLACEMENT_3D('',#34188,#28011,#28012);
#22070=AXIS2_PLACEMENT_3D('',#34194,#28016,#28017);
#22071=AXIS2_PLACEMENT_3D('',#34197,#28018,#28019);
#22072=AXIS2_PLACEMENT_3D('',#34201,#28021,#28022);
#22073=AXIS2_PLACEMENT_3D('',#34203,#28024,#28025);
#22074=AXIS2_PLACEMENT_3D('',#34205,#28026,#28027);
#22075=AXIS2_PLACEMENT_3D('',#34208,#28029,#28030);
#22076=AXIS2_PLACEMENT_3D('',#34209,#28031,#28032);
#22077=AXIS2_PLACEMENT_3D('',#34211,#28033,#28034);
#22078=AXIS2_PLACEMENT_3D('',#34214,#28036,#28037);
#22079=AXIS2_PLACEMENT_3D('',#34215,#28038,#28039);
#22080=AXIS2_PLACEMENT_3D('',#34221,#28043,#28044);
#22081=AXIS2_PLACEMENT_3D('',#34224,#28045,#28046);
#22082=AXIS2_PLACEMENT_3D('',#34228,#28048,#28049);
#22083=AXIS2_PLACEMENT_3D('',#34230,#28051,#28052);
#22084=AXIS2_PLACEMENT_3D('',#34232,#28053,#28054);
#22085=AXIS2_PLACEMENT_3D('',#34235,#28056,#28057);
#22086=AXIS2_PLACEMENT_3D('',#34236,#28058,#28059);
#22087=AXIS2_PLACEMENT_3D('',#34238,#28060,#28061);
#22088=AXIS2_PLACEMENT_3D('',#34241,#28063,#28064);
#22089=AXIS2_PLACEMENT_3D('',#34242,#28065,#28066);
#22090=AXIS2_PLACEMENT_3D('',#34248,#28070,#28071);
#22091=AXIS2_PLACEMENT_3D('',#34251,#28072,#28073);
#22092=AXIS2_PLACEMENT_3D('',#34255,#28075,#28076);
#22093=AXIS2_PLACEMENT_3D('',#34257,#28078,#28079);
#22094=AXIS2_PLACEMENT_3D('',#34259,#28080,#28081);
#22095=AXIS2_PLACEMENT_3D('',#34262,#28083,#28084);
#22096=AXIS2_PLACEMENT_3D('',#34263,#28085,#28086);
#22097=AXIS2_PLACEMENT_3D('',#34265,#28087,#28088);
#22098=AXIS2_PLACEMENT_3D('',#34268,#28090,#28091);
#22099=AXIS2_PLACEMENT_3D('',#34269,#28092,#28093);
#22100=AXIS2_PLACEMENT_3D('',#34275,#28097,#28098);
#22101=AXIS2_PLACEMENT_3D('',#34281,#28102,#28103);
#22102=AXIS2_PLACEMENT_3D('',#34287,#28107,#28108);
#22103=AXIS2_PLACEMENT_3D('',#34293,#28112,#28113);
#22104=AXIS2_PLACEMENT_3D('',#34299,#28117,#28118);
#22105=AXIS2_PLACEMENT_3D('',#34301,#28119,#28120);
#22106=AXIS2_PLACEMENT_3D('',#34304,#28122,#28123);
#22107=AXIS2_PLACEMENT_3D('',#34305,#28124,#28125);
#22108=AXIS2_PLACEMENT_3D('',#34306,#28126,#28127);
#22109=AXIS2_PLACEMENT_3D('',#34307,#28128,#28129);
#22110=AXIS2_PLACEMENT_3D('',#34308,#28130,#28131);
#22111=AXIS2_PLACEMENT_3D('',#34312,#28133,#28134);
#22112=AXIS2_PLACEMENT_3D('',#34315,#28136,#28137);
#22113=AXIS2_PLACEMENT_3D('',#34316,#28138,#28139);
#22114=AXIS2_PLACEMENT_3D('',#34318,#28140,#28141);
#22115=AXIS2_PLACEMENT_3D('',#34320,#28143,#28144);
#22116=AXIS2_PLACEMENT_3D('',#34321,#28145,#28146);
#22117=AXIS2_PLACEMENT_3D('',#34323,#28147,#28148);
#22118=AXIS2_PLACEMENT_3D('',#34325,#28150,#28151);
#22119=AXIS2_PLACEMENT_3D('',#34328,#28153,#28154);
#22120=AXIS2_PLACEMENT_3D('',#34329,#28155,#28156);
#22121=AXIS2_PLACEMENT_3D('',#34331,#28158,#28159);
#22122=AXIS2_PLACEMENT_3D('',#34332,#28160,#28161);
#22123=AXIS2_PLACEMENT_3D('',#34333,#28162,#28163);
#22124=AXIS2_PLACEMENT_3D('',#34337,#28166,#28167);
#22125=AXIS2_PLACEMENT_3D('',#34339,#28168,#28169);
#22126=AXIS2_PLACEMENT_3D('',#34341,#28171,#28172);
#22127=AXIS2_PLACEMENT_3D('',#34343,#28174,#28175);
#22128=AXIS2_PLACEMENT_3D('',#34344,#28176,#28177);
#22129=AXIS2_PLACEMENT_3D('',#34345,#28178,#28179);
#27960=DIRECTION('axis',(0.,0.,1.));
#27961=DIRECTION('refdir',(1.,0.,0.));
#27962=DIRECTION('center_axis',(0.,-1.,0.));
#27963=DIRECTION('ref_axis',(-0.95943850055877,0.,-0.281918008728671));
#27964=DIRECTION('center_axis',(0.,1.,0.));
#27965=DIRECTION('ref_axis',(-0.95943850055113,0.,-0.281918008754672));
#27966=DIRECTION('',(0.,-1.,0.));
#27967=DIRECTION('center_axis',(0.,-1.,0.));
#27968=DIRECTION('ref_axis',(-0.95943850055113,0.,-0.281918008754672));
#27969=DIRECTION('',(0.,1.,0.));
#27970=DIRECTION('center_axis',(0.,-1.,0.));
#27971=DIRECTION('ref_axis',(-0.882269183586981,0.,0.470745247127108));
#27972=DIRECTION('center_axis',(0.,-1.,0.));
#27973=DIRECTION('ref_axis',(-0.882269183586837,0.,0.470745247127378));
#27974=DIRECTION('',(0.,1.,0.));
#27975=DIRECTION('center_axis',(0.,1.,0.));
#27976=DIRECTION('ref_axis',(-0.882269183586837,0.,0.470745247127378));
#27977=DIRECTION('center_axis',(0.,-1.,0.));
#27978=DIRECTION('ref_axis',(-0.235571092936032,0.,0.971857119217081));
#27979=DIRECTION('center_axis',(0.,1.,0.));
#27980=DIRECTION('ref_axis',(-0.235571092964655,0.,0.971857119210143));
#27981=DIRECTION('',(0.,-1.,0.));
#27982=DIRECTION('center_axis',(0.,-1.,0.));
#27983=DIRECTION('ref_axis',(-0.235571092964655,0.,0.971857119210143));
#27984=DIRECTION('center_axis',(0.528694902398929,0.,0.848811934516349));
#27985=DIRECTION('ref_axis',(0.,-1.,0.));
#27986=DIRECTION('',(-0.84881193451618,0.,0.528694902399201));
#27987=DIRECTION('',(0.,1.,0.));
#27988=DIRECTION('',(0.84881193451618,0.,-0.528694902399201));
#27989=DIRECTION('center_axis',(0.,-1.,0.));
#27990=DIRECTION('ref_axis',(-0.9880280553808,0.,-0.154274306935522));
#27991=DIRECTION('center_axis',(0.,1.,0.));
#27992=DIRECTION('ref_axis',(-0.988028055375654,0.,-0.154274306968473));
#27993=DIRECTION('',(0.,-1.,0.));
#27994=DIRECTION('center_axis',(0.,-1.,0.));
#27995=DIRECTION('ref_axis',(-0.988028055375654,0.,-0.154274306968473));
#27996=DIRECTION('',(0.,1.,0.));
#27997=DIRECTION('center_axis',(0.,-1.,0.));
#27998=DIRECTION('ref_axis',(-0.813276663802591,0.,0.581877193327017));
#27999=DIRECTION('center_axis',(0.,-1.,0.));
#28000=DIRECTION('ref_axis',(-0.813276663802491,0.,0.581877193327157));
#28001=DIRECTION('',(0.,1.,0.));
#28002=DIRECTION('center_axis',(0.,1.,0.));
#28003=DIRECTION('ref_axis',(-0.813276663802491,0.,0.581877193327157));
#28004=DIRECTION('center_axis',(0.,-1.,0.));
#28005=DIRECTION('ref_axis',(-0.106702940426287,0.,0.994290944595386));
#28006=DIRECTION('center_axis',(0.,1.,0.));
#28007=DIRECTION('ref_axis',(-0.106702940461588,0.,0.994290944591597));
#28008=DIRECTION('',(0.,-1.,0.));
#28009=DIRECTION('center_axis',(0.,-1.,0.));
#28010=DIRECTION('ref_axis',(-0.106702940461588,0.,0.994290944591597));
#28011=DIRECTION('center_axis',(0.634964033941301,0.,0.772541698292714));
#28012=DIRECTION('ref_axis',(0.,-1.,0.));
#28013=DIRECTION('',(-0.772541698292626,0.,0.634964033941407));
#28014=DIRECTION('',(0.,1.,0.));
#28015=DIRECTION('',(0.772541698292626,0.,-0.634964033941407));
#28016=DIRECTION('center_axis',(0.,-1.,0.));
#28017=DIRECTION('ref_axis',(-0.999712176242133,0.,-0.0239909289777924));
#28018=DIRECTION('center_axis',(0.,1.,0.));
#28019=DIRECTION('ref_axis',(-0.999712176241197,0.,-0.0239909290168101));
#28020=DIRECTION('',(0.,-1.,0.));
#28021=DIRECTION('center_axis',(0.,-1.,0.));
#28022=DIRECTION('ref_axis',(-0.999712176241197,0.,-0.0239909290168101));
#28023=DIRECTION('',(0.,1.,0.));
#28024=DIRECTION('center_axis',(0.,-1.,0.));
#28025=DIRECTION('ref_axis',(-0.730368754817649,0.,0.683053059422266));
#28026=DIRECTION('center_axis',(0.,-1.,0.));
#28027=DIRECTION('ref_axis',(-0.730368754817625,0.,0.683053059422291));
#28028=DIRECTION('',(0.,1.,0.));
#28029=DIRECTION('center_axis',(0.,1.,0.));
#28030=DIRECTION('ref_axis',(-0.730368754817625,0.,0.683053059422291));
#28031=DIRECTION('center_axis',(0.,-1.,0.));
#28032=DIRECTION('ref_axis',(0.0239909289777986,0.,0.999712176242133));
#28033=DIRECTION('center_axis',(0.,1.,0.));
#28034=DIRECTION('ref_axis',(0.0239909290168162,0.,0.999712176241197));
#28035=DIRECTION('',(0.,-1.,0.));
#28036=DIRECTION('center_axis',(0.,-1.,0.));
#28037=DIRECTION('ref_axis',(0.0239909290168162,0.,0.999712176241197));
#28038=DIRECTION('center_axis',(0.730368754817649,0.,0.683053059422266));
#28039=DIRECTION('ref_axis',(0.,-1.,0.));
#28040=DIRECTION('',(-0.683053059422301,0.,0.730368754817616));
#28041=DIRECTION('',(0.,1.,0.));
#28042=DIRECTION('',(0.683053059422301,0.,-0.730368754817616));
#28043=DIRECTION('center_axis',(0.,-1.,0.));
#28044=DIRECTION('ref_axis',(-0.994290944595386,0.,0.106702940426287));
#28045=DIRECTION('center_axis',(0.,1.,0.));
#28046=DIRECTION('ref_axis',(-0.994290944591597,0.,0.106702940461588));
#28047=DIRECTION('',(0.,-1.,0.));
#28048=DIRECTION('center_axis',(0.,-1.,0.));
#28049=DIRECTION('ref_axis',(-0.994290944591597,0.,0.106702940461588));
#28050=DIRECTION('',(0.,1.,0.));
#28051=DIRECTION('center_axis',(0.,-1.,0.));
#28052=DIRECTION('ref_axis',(-0.634964033941301,0.,0.772541698292714));
#28053=DIRECTION('center_axis',(0.,-1.,0.));
#28054=DIRECTION('ref_axis',(-0.63496403394138,0.,0.772541698292649));
#28055=DIRECTION('',(0.,1.,0.));
#28056=DIRECTION('center_axis',(0.,1.,0.));
#28057=DIRECTION('ref_axis',(-0.63496403394138,0.,0.772541698292649));
#28058=DIRECTION('center_axis',(0.,-1.,0.));
#28059=DIRECTION('ref_axis',(0.15427430693553,0.,0.988028055380798));
#28060=DIRECTION('center_axis',(0.,1.,0.));
#28061=DIRECTION('ref_axis',(0.154274306968481,0.,0.988028055375653));
#28062=DIRECTION('',(0.,-1.,0.));
#28063=DIRECTION('center_axis',(0.,-1.,0.));
#28064=DIRECTION('ref_axis',(0.154274306968481,0.,0.988028055375653));
#28065=DIRECTION('center_axis',(0.813276663802591,0.,0.581877193327018));
#28066=DIRECTION('ref_axis',(0.,-1.,0.));
#28067=DIRECTION('',(-0.581877193327205,0.,0.813276663802457));
#28068=DIRECTION('',(0.,1.,0.));
#28069=DIRECTION('',(0.581877193327205,0.,-0.813276663802457));
#28070=DIRECTION('center_axis',(0.,-1.,0.));
#28071=DIRECTION('ref_axis',(-0.971857119217081,0.,0.235571092936033));
#28072=DIRECTION('center_axis',(0.,1.,0.));
#28073=DIRECTION('ref_axis',(-0.971857119210143,0.,0.235571092964656));
#28074=DIRECTION('',(0.,-1.,0.));
#28075=DIRECTION('center_axis',(0.,-1.,0.));
#28076=DIRECTION('ref_axis',(-0.971857119210143,0.,0.235571092964656));
#28077=DIRECTION('',(0.,1.,0.));
#28078=DIRECTION('center_axis',(0.,-1.,0.));
#28079=DIRECTION('ref_axis',(-0.528694902398929,0.,0.848811934516349));
#28080=DIRECTION('center_axis',(0.,-1.,0.));
#28081=DIRECTION('ref_axis',(-0.528694902399131,0.,0.848811934516223));
#28082=DIRECTION('',(0.,1.,0.));
#28083=DIRECTION('center_axis',(0.,1.,0.));
#28084=DIRECTION('ref_axis',(-0.528694902399131,0.,0.848811934516223));
#28085=DIRECTION('center_axis',(0.,-1.,0.));
#28086=DIRECTION('ref_axis',(0.281918008728669,0.,0.959438500558771));
#28087=DIRECTION('center_axis',(0.,1.,0.));
#28088=DIRECTION('ref_axis',(0.28191800875467,0.,0.959438500551131));
#28089=DIRECTION('',(0.,-1.,0.));
#28090=DIRECTION('center_axis',(0.,-1.,0.));
#28091=DIRECTION('ref_axis',(0.28191800875467,0.,0.959438500551131));
#28092=DIRECTION('center_axis',(0.882269183586981,0.,0.470745247127108));
#28093=DIRECTION('ref_axis',(0.,-1.,0.));
#28094=DIRECTION('',(-0.470745247127471,0.,0.882269183586787));
#28095=DIRECTION('',(0.,1.,0.));
#28096=DIRECTION('',(0.470745247127471,0.,-0.882269183586787));
#28097=DIRECTION('center_axis',(-0.848811934516349,0.,-0.528694902398929));
#28098=DIRECTION('ref_axis',(-0.528694902398929,0.,0.848811934516349));
#28099=DIRECTION('',(-0.528694902399201,0.,0.84881193451618));
#28100=DIRECTION('',(0.,-1.,0.));
#28101=DIRECTION('',(0.528694902399201,0.,-0.84881193451618));
#28102=DIRECTION('center_axis',(-0.772541698292714,0.,-0.634964033941301));
#28103=DIRECTION('ref_axis',(-0.634964033941301,0.,0.772541698292714));
#28104=DIRECTION('',(-0.634964033941407,0.,0.772541698292626));
#28105=DIRECTION('',(0.,-1.,0.));
#28106=DIRECTION('',(0.634964033941407,0.,-0.772541698292626));
#28107=DIRECTION('center_axis',(-0.581877193327018,0.,-0.813276663802591));
#28108=DIRECTION('ref_axis',(-0.813276663802591,0.,0.581877193327018));
#28109=DIRECTION('',(-0.813276663802456,0.,0.581877193327206));
#28110=DIRECTION('',(0.,-1.,0.));
#28111=DIRECTION('',(0.813276663802456,0.,-0.581877193327206));
#28112=DIRECTION('center_axis',(-0.470745247127108,0.,-0.882269183586981));
#28113=DIRECTION('ref_axis',(-0.882269183586981,0.,0.470745247127108));
#28114=DIRECTION('',(-0.882269183586787,0.,0.470745247127471));
#28115=DIRECTION('',(0.,-1.,0.));
#28116=DIRECTION('',(0.882269183586787,0.,-0.470745247127471));
#28117=DIRECTION('center_axis',(0.,1.,0.));
#28118=DIRECTION('ref_axis',(0.902585284349861,0.,-0.430511096808295));
#28119=DIRECTION('center_axis',(0.,-1.,0.));
#28120=DIRECTION('ref_axis',(0.902585284349705,0.,-0.430511096808622));
#28121=DIRECTION('',(0.,-1.,0.));
#28122=DIRECTION('center_axis',(0.,1.,0.));
#28123=DIRECTION('ref_axis',(0.902585284349705,0.,-0.430511096808622));
#28124=DIRECTION('center_axis',(0.,1.,0.));
#28125=DIRECTION('ref_axis',(0.902585284349861,0.,-0.430511096808295));
#28126=DIRECTION('center_axis',(0.,1.,0.));
#28127=DIRECTION('ref_axis',(0.902585284349705,0.,-0.430511096808622));
#28128=DIRECTION('center_axis',(0.,-1.,0.));
#28129=DIRECTION('ref_axis',(0.902585284349705,0.,-0.430511096808622));
#28130=DIRECTION('center_axis',(0.,1.,0.));
#28131=DIRECTION('ref_axis',(1.,0.,0.));
#28132=DIRECTION('',(-0.430511096808717,0.,0.902585284349659));
#28133=DIRECTION('center_axis',(0.,-1.,0.));
#28134=DIRECTION('ref_axis',(-0.902585284349714,0.,0.430511096808602));
#28135=DIRECTION('',(0.902585284349659,0.,-0.430511096808717));
#28136=DIRECTION('center_axis',(0.,1.,0.));
#28137=DIRECTION('ref_axis',(0.902585284349705,0.,-0.430511096808622));
#28138=DIRECTION('center_axis',(0.,1.,0.));
#28139=DIRECTION('ref_axis',(0.902585284349705,0.,-0.430511096808622));
#28140=DIRECTION('center_axis',(0.,1.,0.));
#28141=DIRECTION('ref_axis',(0.902585284349705,0.,-0.430511096808622));
#28142=DIRECTION('',(-0.730368754817616,0.,0.683053059422301));
#28143=DIRECTION('center_axis',(0.,1.,0.));
#28144=DIRECTION('ref_axis',(0.902585284349705,0.,-0.430511096808622));
#28145=DIRECTION('center_axis',(0.,1.,0.));
#28146=DIRECTION('ref_axis',(0.902585284349861,0.,-0.430511096808295));
#28147=DIRECTION('center_axis',(0.,-1.,0.));
#28148=DIRECTION('ref_axis',(0.902585284349705,0.,-0.430511096808622));
#28149=DIRECTION('',(0.,-1.,0.));
#28150=DIRECTION('center_axis',(0.,1.,0.));
#28151=DIRECTION('ref_axis',(0.902585284349861,0.,-0.430511096808295));
#28152=DIRECTION('',(0.,1.,0.));
#28153=DIRECTION('center_axis',(0.,-1.,0.));
#28154=DIRECTION('ref_axis',(0.902585284349705,0.,-0.430511096808622));
#28155=DIRECTION('center_axis',(-0.683053059422266,0.,-0.730368754817649));
#28156=DIRECTION('ref_axis',(-0.730368754817649,0.,0.683053059422266));
#28157=DIRECTION('',(0.730368754817616,0.,-0.683053059422301));
#28158=DIRECTION('center_axis',(0.,1.,0.));
#28159=DIRECTION('ref_axis',(0.902585284349861,0.,-0.430511096808295));
#28160=DIRECTION('center_axis',(0.,-1.,0.));
#28161=DIRECTION('ref_axis',(0.902585284349705,0.,-0.430511096808622));
#28162=DIRECTION('center_axis',(0.902585284349863,0.,0.430511096808291));
#28163=DIRECTION('ref_axis',(0.,-1.,0.));
#28164=DIRECTION('',(0.430511096808717,0.,-0.902585284349659));
#28165=DIRECTION('',(0.,1.,0.));
#28166=DIRECTION('center_axis',(0.,1.,0.));
#28167=DIRECTION('ref_axis',(-0.902585284349861,0.,0.430511096808295));
#28168=DIRECTION('center_axis',(0.,1.,0.));
#28169=DIRECTION('ref_axis',(-0.902585284349714,0.,0.430511096808602));
#28170=DIRECTION('',(0.,1.,0.));
#28171=DIRECTION('center_axis',(-0.430511096808291,0.,-0.902585284349863));
#28172=DIRECTION('ref_axis',(-0.902585284349863,0.,0.430511096808291));
#28173=DIRECTION('',(-0.902585284349659,0.,0.430511096808717));
#28174=DIRECTION('center_axis',(0.,1.,0.));
#28175=DIRECTION('ref_axis',(0.902585284349861,0.,-0.430511096808295));
#28176=DIRECTION('center_axis',(0.,-1.,0.));
#28177=DIRECTION('ref_axis',(0.902585284349705,0.,-0.430511096808622));
#28178=DIRECTION('center_axis',(0.,1.,0.));
#28179=DIRECTION('ref_axis',(1.,0.,0.));
#34139=CARTESIAN_POINT('',(0.,0.,0.));
#34140=CARTESIAN_POINT('Origin',(-0.0115261780187742,-0.008,0.00643329000430777));
#34141=CARTESIAN_POINT('',(-0.011643864330556,-0.008,0.00621272270841102));
#34142=CARTESIAN_POINT('',(-0.0117444768448874,-0.008,0.00655513261802572));
#34143=CARTESIAN_POINT('Origin',(-0.0115261780187842,-0.00799999999999,
0.00643329000431777));
#34144=CARTESIAN_POINT('',(-0.0117444768448874,-0.024,0.00655513261802572));
#34145=CARTESIAN_POINT('',(-0.0117444768448974,-0.00799999999999,0.00655513261803572));
#34146=CARTESIAN_POINT('',(-0.011643864330556,-0.024,0.00621272270841102));
#34147=CARTESIAN_POINT('Origin',(-0.0115261780187842,-0.02400000000001,
0.00643329000431777));
#34148=CARTESIAN_POINT('',(-0.011643864330566,-0.00799999999999,0.00621272270842102));
#34149=CARTESIAN_POINT('Origin',(-4.44089209850063E-17,-0.008,6.72997231505748E-33));
#34150=CARTESIAN_POINT('',(-0.0115491497948299,-0.008,0.00689344899281771));
#34151=CARTESIAN_POINT('Origin',(-4.44089209850063E-17,-0.00799999999999,
6.72997231505748E-33));
#34152=CARTESIAN_POINT('',(-0.0115491497948299,-0.024,0.00689344899281771));
#34153=CARTESIAN_POINT('',(-0.0115491497948399,-0.00799999999999,0.00689344899282771));
#34154=CARTESIAN_POINT('Origin',(-4.44089209850063E-17,-0.02400000000001,
6.72997231505748E-33));
#34155=CARTESIAN_POINT('Origin',(-0.0113344815830301,-0.008,0.00676531797064638));
#34156=CARTESIAN_POINT('',(-0.0112023078574304,-0.008,0.00697752095427546));
#34157=CARTESIAN_POINT('Origin',(-0.0113344815830401,-0.00799999999999,
0.00676531797065638));
#34158=CARTESIAN_POINT('',(-0.0112023078574304,-0.024,0.00697752095427546));
#34159=CARTESIAN_POINT('',(-0.0112023078574404,-0.00799999999999,0.00697752095428546));
#34160=CARTESIAN_POINT('Origin',(-0.0113344815830401,-0.02400000000001,
0.00676531797065638));
#34161=CARTESIAN_POINT('Origin',(-0.0110345551487125,-0.008,0.00687303373118608));
#34162=CARTESIAN_POINT('',(-0.0110345551487125,-0.008,0.00687303373118608));
#34163=CARTESIAN_POINT('',(-0.0108205542946554,-0.00799999999999,0.00673974017575289));
#34164=CARTESIAN_POINT('',(-0.0110345551487125,-0.024,0.00687303373118608));
#34165=CARTESIAN_POINT('',(-0.0110345551487225,-0.016,0.00687303373119607));
#34166=CARTESIAN_POINT('',(-0.0108205542946554,-0.02400000000001,0.00673974017575289));
#34167=CARTESIAN_POINT('Origin',(-0.0105878571202838,-0.008,0.00788272044413949));
#34168=CARTESIAN_POINT('',(-0.0107333264186156,-0.008,0.00767940127818885));
#34169=CARTESIAN_POINT('',(-0.0107883847172589,-0.008,0.00803201439194517));
#34170=CARTESIAN_POINT('Origin',(-0.0105878571202938,-0.00799999999999,
0.00788272044414949));
#34171=CARTESIAN_POINT('',(-0.0107883847172589,-0.024,0.00803201439194517));
#34172=CARTESIAN_POINT('',(-0.0107883847172689,-0.00799999999999,0.00803201439195517));
#34173=CARTESIAN_POINT('',(-0.0107333264186156,-0.024,0.00767940127818885));
#34174=CARTESIAN_POINT('Origin',(-0.0105878571202938,-0.02400000000001,
0.00788272044414949));
#34175=CARTESIAN_POINT('',(-0.0107333264186256,-0.00799999999999,0.00767940127819885));
#34176=CARTESIAN_POINT('Origin',(-4.44089209850063E-17,-0.008,6.72997231505748E-33));
#34177=CARTESIAN_POINT('',(-0.0105505695690249,-0.008,0.00834194112716973));
#34178=CARTESIAN_POINT('Origin',(-4.44089209850063E-17,-0.00799999999999,
6.72997231505748E-33));
#34179=CARTESIAN_POINT('',(-0.0105505695690249,-0.024,0.00834194112716973));
#34180=CARTESIAN_POINT('',(-0.0105505695690349,-0.00799999999999,0.00834194112717973));
#34181=CARTESIAN_POINT('Origin',(-4.44089209850063E-17,-0.02400000000001,
6.72997231505748E-33));
#34182=CARTESIAN_POINT('Origin',(-0.010354462327965,-0.008,0.00818688645937847));
#34183=CARTESIAN_POINT('',(-0.0101957213194796,-0.008,0.00838002188395165));
#34184=CARTESIAN_POINT('Origin',(-0.010354462327975,-0.00799999999999,0.00818688645938847));
#34185=CARTESIAN_POINT('',(-0.0101957213194796,-0.024,0.00838002188395165));
#34186=CARTESIAN_POINT('',(-0.0101957213194896,-0.00799999999999,0.00838002188396165));
#34187=CARTESIAN_POINT('Origin',(-0.010354462327975,-0.02400000000001,0.00818688645938847));
#34188=CARTESIAN_POINT('Origin',(-0.0100430420778053,-0.008,0.00825453244123692));
#34189=CARTESIAN_POINT('',(-0.0100430420778053,-0.008,0.00825453244123692));
#34190=CARTESIAN_POINT('',(-0.00995338570524494,-0.00799999999999,0.00818084247458021));
#34191=CARTESIAN_POINT('',(-0.0100430420778053,-0.024,0.00825453244123692));
#34192=CARTESIAN_POINT('',(-0.0100430420778153,-0.016,0.00825453244124691));
#34193=CARTESIAN_POINT('',(-0.00995338570524494,-0.02400000000001,0.00818084247458021));
#34194=CARTESIAN_POINT('Origin',(-0.00946837505095689,-0.008,0.00919727535166899));
#34195=CARTESIAN_POINT('',(-0.00963913831581246,-0.008,0.00901468316296458));
#34196=CARTESIAN_POINT('',(-0.00964770033601289,-0.008,0.00937146617272333));
#34197=CARTESIAN_POINT('Origin',(-0.00946837505096689,-0.00799999999999,
0.00919727535167899));
#34198=CARTESIAN_POINT('',(-0.00964770033601289,-0.024,0.00937146617272333));
#34199=CARTESIAN_POINT('',(-0.0096477003360229,-0.00799999999999,0.00937146617273333));
#34200=CARTESIAN_POINT('',(-0.00963913831581246,-0.024,0.00901468316296458));
#34201=CARTESIAN_POINT('Origin',(-0.00946837505096689,-0.02400000000001,
0.00919727535167899));
#34202=CARTESIAN_POINT('',(-0.00963913831582247,-0.00799999999999,0.00901468316297458));
#34203=CARTESIAN_POINT('Origin',(-4.44089209850063E-17,-0.008,6.72997231505748E-33));
#34204=CARTESIAN_POINT('',(-0.00937146617272338,-0.008,0.00964770033601285));
#34205=CARTESIAN_POINT('Origin',(-4.44089209850063E-17,-0.00799999999999,
6.72997231505748E-33));
#34206=CARTESIAN_POINT('',(-0.00937146617272338,-0.024,0.00964770033601285));
#34207=CARTESIAN_POINT('',(-0.00937146617273337,-0.00799999999999,0.00964770033602285));
#34208=CARTESIAN_POINT('Origin',(-4.44089209850063E-17,-0.02400000000001,
6.72997231505748E-33));
#34209=CARTESIAN_POINT('Origin',(-0.00919727535166904,-0.008,0.00946837505095685));
#34210=CARTESIAN_POINT('',(-0.00901468316296463,-0.008,0.00963913831581242));
#34211=CARTESIAN_POINT('Origin',(-0.00919727535167904,-0.00799999999999,
0.00946837505096685));
#34212=CARTESIAN_POINT('',(-0.00901468316296463,-0.024,0.00963913831581242));
#34213=CARTESIAN_POINT('',(-0.00901468316297463,-0.00799999999999,0.00963913831582242));
#34214=CARTESIAN_POINT('Origin',(-0.00919727535167904,-0.02400000000001,
0.00946837505096685));
#34215=CARTESIAN_POINT('Origin',(-0.0088796897724895,-0.008,0.00949479381262943));
#34216=CARTESIAN_POINT('',(-0.0088796897724895,-0.008,0.00949479381262943));
#34217=CARTESIAN_POINT('',(-0.00881874742507032,-0.00799999999999,0.00942962993438206));
#34218=CARTESIAN_POINT('',(-0.0088796897724895,-0.024,0.00949479381262943));
#34219=CARTESIAN_POINT('',(-0.00887968977249951,-0.016,0.00949479381263943));
#34220=CARTESIAN_POINT('',(-0.00881874742507032,-0.02400000000001,0.00942962993438206));
#34221=CARTESIAN_POINT('Origin',(-0.00818688645937852,-0.008,0.010354462327965));
#34222=CARTESIAN_POINT('',(-0.00838002188395169,-0.008,0.0101957213194796));
#34223=CARTESIAN_POINT('',(-0.00834194112716978,-0.008,0.0105505695690249));
#34224=CARTESIAN_POINT('Origin',(-0.00818688645938851,-0.00799999999999,
0.010354462327975));
#34225=CARTESIAN_POINT('',(-0.00834194112716978,-0.024,0.0105505695690249));
#34226=CARTESIAN_POINT('',(-0.00834194112717978,-0.00799999999999,0.0105505695690349));
#34227=CARTESIAN_POINT('',(-0.00838002188395169,-0.024,0.0101957213194796));
#34228=CARTESIAN_POINT('Origin',(-0.00818688645938851,-0.02400000000001,
0.010354462327975));
#34229=CARTESIAN_POINT('',(-0.0083800218839617,-0.00799999999999,0.0101957213194896));
#34230=CARTESIAN_POINT('Origin',(-4.44089209850063E-17,-0.008,6.72997231505748E-33));
#34231=CARTESIAN_POINT('',(-0.00803201439194522,-0.008,0.0107883847172589));
#34232=CARTESIAN_POINT('Origin',(-4.44089209850063E-17,-0.00799999999999,
6.72997231505748E-33));
#34233=CARTESIAN_POINT('',(-0.00803201439194522,-0.024,0.0107883847172589));
#34234=CARTESIAN_POINT('',(-0.00803201439195521,-0.00799999999999,0.0107883847172689));
#34235=CARTESIAN_POINT('Origin',(-4.44089209850063E-17,-0.02400000000001,
6.72997231505748E-33));
#34236=CARTESIAN_POINT('Origin',(-0.00788272044413954,-0.008,0.0105878571202839));
#34237=CARTESIAN_POINT('',(-0.00767940127818889,-0.008,0.0107333264186156));
#34238=CARTESIAN_POINT('Origin',(-0.00788272044414953,-0.00799999999999,
0.0105878571202939));
#34239=CARTESIAN_POINT('',(-0.00767940127818889,-0.024,0.0107333264186156));
#34240=CARTESIAN_POINT('',(-0.00767940127819889,-0.00799999999999,0.0107333264186256));
#34241=CARTESIAN_POINT('Origin',(-0.00788272044414953,-0.02400000000001,
0.0105878571202939));
#34242=CARTESIAN_POINT('Origin',(-0.00756440351325127,-0.008,0.0105725966294337));
#34243=CARTESIAN_POINT('',(-0.00756440351325127,-0.008,0.0105725966294337));
#34244=CARTESIAN_POINT('',(-0.00746427554955181,-0.00799999999999,0.0104326500269426));
#34245=CARTESIAN_POINT('',(-0.00756440351325127,-0.024,0.0105725966294337));
#34246=CARTESIAN_POINT('',(-0.00756440351326127,-0.016,0.0105725966294437));
#34247=CARTESIAN_POINT('',(-0.00746427554955181,-0.02400000000001,0.0104326500269426));
#34248=CARTESIAN_POINT('Origin',(-0.00676531797064642,-0.008,0.0113344815830301));
#34249=CARTESIAN_POINT('',(-0.00697752095427551,-0.008,0.0112023078574304));
#34250=CARTESIAN_POINT('',(-0.00689344899281775,-0.008,0.01154914979483));
#34251=CARTESIAN_POINT('Origin',(-0.00676531797065643,-0.00799999999999,
0.0113344815830401));
#34252=CARTESIAN_POINT('',(-0.00689344899281775,-0.024,0.01154914979483));
#34253=CARTESIAN_POINT('',(-0.00689344899282776,-0.00799999999999,0.0115491497948399));
#34254=CARTESIAN_POINT('',(-0.00697752095427551,-0.024,0.0112023078574304));
#34255=CARTESIAN_POINT('Origin',(-0.00676531797065643,-0.02400000000001,
0.0113344815830401));
#34256=CARTESIAN_POINT('',(-0.00697752095428551,-0.00799999999999,0.0112023078574404));
#34257=CARTESIAN_POINT('Origin',(-4.44089209850063E-17,-0.008,6.72997231505748E-33));
#34258=CARTESIAN_POINT('',(-0.00655513261802576,-0.008,0.0117444768448874));
#34259=CARTESIAN_POINT('Origin',(-4.44089209850063E-17,-0.00799999999999,
6.72997231505748E-33));
#34260=CARTESIAN_POINT('',(-0.00655513261802576,-0.024,0.0117444768448874));
#34261=CARTESIAN_POINT('',(-0.00655513261803576,-0.00799999999999,0.0117444768448974));
#34262=CARTESIAN_POINT('Origin',(-4.44089209850063E-17,-0.02400000000001,
6.72997231505748E-33));
#34263=CARTESIAN_POINT('Origin',(-0.00643329000430782,-0.008,0.0115261780187742));
#34264=CARTESIAN_POINT('',(-0.00621272270841107,-0.008,0.011643864330556));
#34265=CARTESIAN_POINT('Origin',(-0.00643329000431782,-0.00799999999999,
0.0115261780187842));
#34266=CARTESIAN_POINT('',(-0.00621272270841107,-0.024,0.011643864330556));
#34267=CARTESIAN_POINT('',(-0.00621272270842108,-0.00799999999999,0.011643864330566));
#34268=CARTESIAN_POINT('Origin',(-0.00643329000431782,-0.02400000000001,
0.0115261780187842));
#34269=CARTESIAN_POINT('Origin',(-0.00611968821265244,-0.008,0.0114694993866308));
#34270=CARTESIAN_POINT('',(-0.00611968821265244,-0.008,0.0114694993866308));
#34271=CARTESIAN_POINT('',(-0.00594871026243943,-0.00799999999999,0.0111490530784194));
#34272=CARTESIAN_POINT('',(-0.00611968821265244,-0.024,0.0114694993866308));
#34273=CARTESIAN_POINT('',(-0.00611968821266244,-0.016,0.0114694993866408));
#34274=CARTESIAN_POINT('',(-0.00594871026243943,-0.02400000000001,0.0111490530784194));
#34275=CARTESIAN_POINT('Origin',(-0.00711094643726563,-0.008,0.0114165205192449));
#34276=CARTESIAN_POINT('',(-0.00687303373118612,-0.024,0.0110345551487125));
#34277=CARTESIAN_POINT('',(-0.00685869652879269,-0.02400000000001,0.0110115369799216));
#34278=CARTESIAN_POINT('',(-0.00687303373118612,-0.008,0.0110345551487125));
#34279=CARTESIAN_POINT('',(-0.00687303373119612,-0.016,0.0110345551487225));
#34280=CARTESIAN_POINT('',(-0.00685869652879269,-0.00799999999999,0.0110115369799216));
#34281=CARTESIAN_POINT('Origin',(-0.00854026625651055,-0.008,0.010390685842037));
#34282=CARTESIAN_POINT('',(-0.00825453244123696,-0.024,0.0100430420778053));
#34283=CARTESIAN_POINT('',(-0.00832370938221705,-0.02400000000001,0.0101272075873608));
#34284=CARTESIAN_POINT('',(-0.00825453244123696,-0.008,0.0100430420778053));
#34285=CARTESIAN_POINT('',(-0.00825453244124696,-0.016,0.0100430420778153));
#34286=CARTESIAN_POINT('',(-0.00832370938221705,-0.00799999999999,0.0101272075873608));
#34287=CARTESIAN_POINT('Origin',(-0.0109385711281449,-0.008,0.00782624825024839));
#34288=CARTESIAN_POINT('',(-0.0105725966294337,-0.024,0.00756440351325123));
#34289=CARTESIAN_POINT('',(-0.0106156372762982,-0.02400000000001,0.00759519791805035));
#34290=CARTESIAN_POINT('',(-0.0105725966294337,-0.008,0.00756440351325123));
#34291=CARTESIAN_POINT('',(-0.0105725966294437,-0.016,0.00756440351326123));
#34292=CARTESIAN_POINT('',(-0.0106156372762982,-0.00799999999999,0.00759519791805035));
#34293=CARTESIAN_POINT('Origin',(-0.0118665205192449,-0.008,0.0063315235738596));
#34294=CARTESIAN_POINT('',(-0.0114694993866308,-0.024,0.0061196882126524));
#34295=CARTESIAN_POINT('',(-0.0113475636447265,-0.02400000000001,0.00605462794304299));
#34296=CARTESIAN_POINT('',(-0.0114694993866308,-0.008,0.0061196882126524));
#34297=CARTESIAN_POINT('',(-0.0114694993866408,-0.016,0.0061196882126624));
#34298=CARTESIAN_POINT('',(-0.0113475636447265,-0.00799999999999,0.00605462794304299));
#34299=CARTESIAN_POINT('Origin',(-4.44089209850063E-17,-0.016,6.72997231505748E-33));
#34300=CARTESIAN_POINT('',(-0.00559664425850789,-0.008,0.0117336086965482));
#34301=CARTESIAN_POINT('Origin',(-4.44089209850063E-17,-0.00799999999999,
6.72997231505748E-33));
#34302=CARTESIAN_POINT('',(-0.00559664425850789,-0.024,0.0117336086965482));
#34303=CARTESIAN_POINT('',(-0.00559664425851789,-0.016,0.0117336086965582));
#34304=CARTESIAN_POINT('Origin',(-4.44089209850063E-17,-0.02400000000001,
6.72997231505748E-33));
#34305=CARTESIAN_POINT('Origin',(-4.44089209850063E-17,-0.016,6.72997231505748E-33));
#34306=CARTESIAN_POINT('Origin',(-4.44089209850063E-17,-0.02400000000001,
6.72997231505748E-33));
#34307=CARTESIAN_POINT('Origin',(-4.44089209850063E-17,-0.00799999999999,
6.72997231505748E-33));
#34308=CARTESIAN_POINT('Origin',(-0.0090712898554855,-0.024,0.00907128985548545));
#34309=CARTESIAN_POINT('',(-0.00598410424563535,-0.024,0.0125459354524631));
#34310=CARTESIAN_POINT('',(-0.00598410424564535,-0.02400000000001,0.0125459354524731));
#34311=CARTESIAN_POINT('',(-0.0125459354524631,-0.024,0.0059841042456353));
#34312=CARTESIAN_POINT('Origin',(-4.44089209850063E-17,-0.02400000000001,
6.72997231505748E-33));
#34313=CARTESIAN_POINT('',(-0.0117336086965482,-0.024,0.00559664425850784));
#34314=CARTESIAN_POINT('',(-0.0117336086965582,-0.02400000000001,0.00559664425851784));
#34315=CARTESIAN_POINT('Origin',(-4.44089209850063E-17,-0.02400000000001,
6.72997231505748E-33));
#34316=CARTESIAN_POINT('Origin',(-4.44089209850063E-17,-0.02400000000001,
6.72997231505748E-33));
#34317=CARTESIAN_POINT('',(-0.00949479381262948,-0.024,0.00887968977248946));
#34318=CARTESIAN_POINT('Origin',(-4.44089209850063E-17,-0.02400000000001,
6.72997231505748E-33));
#34319=CARTESIAN_POINT('',(-0.00959396290421607,-0.02400000000001,0.00897243436344028));
#34320=CARTESIAN_POINT('Origin',(-4.44089209850063E-17,-0.02400000000001,
6.72997231505748E-33));
#34321=CARTESIAN_POINT('Origin',(-4.44089209850063E-17,-0.016,6.72997231505748E-33));
#34322=CARTESIAN_POINT('',(-0.00949479381262948,-0.008,0.00887968977248946));
#34323=CARTESIAN_POINT('Origin',(-4.44089209850063E-17,-0.00799999999999,
6.72997231505748E-33));
#34324=CARTESIAN_POINT('',(-0.00949479381263948,-0.016,0.00887968977249946));
#34325=CARTESIAN_POINT('Origin',(-4.44089209850063E-17,-0.016,6.72997231505748E-33));
#34326=CARTESIAN_POINT('',(-0.0117336086965482,-0.008,0.00559664425850784));
#34327=CARTESIAN_POINT('',(-0.0117336086965582,-0.016,0.00559664425851784));
#34328=CARTESIAN_POINT('Origin',(-4.44089209850063E-17,-0.00799999999999,
6.72997231505748E-33));
#34329=CARTESIAN_POINT('Origin',(-0.00982345975229741,-0.008,0.00918706364922948));
#34330=CARTESIAN_POINT('',(-0.00959396290421607,-0.00799999999999,0.00897243436344028));
#34331=CARTESIAN_POINT('Origin',(-4.44089209850063E-17,-0.016,6.72997231505748E-33));
#34332=CARTESIAN_POINT('Origin',(-4.44089209850063E-17,-0.00799999999999,
6.72997231505748E-33));
#34333=CARTESIAN_POINT('Origin',(-0.00598410424563535,-0.016,0.0125459354524631));
#34334=CARTESIAN_POINT('',(-0.00598410424563535,-0.008,0.0125459354524631));
#34335=CARTESIAN_POINT('',(-0.00598410424564535,-0.00799999999999,0.0125459354524731));
#34336=CARTESIAN_POINT('',(-0.00598410424564535,-0.016,0.0125459354524731));
#34337=CARTESIAN_POINT('Origin',(-4.44089209850063E-17,-0.016,6.72997231505748E-33));
#34338=CARTESIAN_POINT('',(-0.0125459354524631,-0.008,0.0059841042456353));
#34339=CARTESIAN_POINT('Origin',(-4.44089209850063E-17,-0.00799999999999,
6.72997231505748E-33));
#34340=CARTESIAN_POINT('',(-0.0125459354524731,-0.016,0.0059841042456453));
#34341=CARTESIAN_POINT('Origin',(-0.0117336086965482,-0.016,0.00559664425850784));
#34342=CARTESIAN_POINT('',(-0.0117336086965582,-0.00799999999999,0.00559664425851784));
#34343=CARTESIAN_POINT('Origin',(-4.44089209850063E-17,-0.016,6.72997231505748E-33));
#34344=CARTESIAN_POINT('Origin',(-4.44089209850063E-17,-0.00799999999999,
6.72997231505748E-33));
#34345=CARTESIAN_POINT('Origin',(-0.0090712898554855,-0.008,0.00907128985548545));
#34837=UNCERTAINTY_MEASURE_WITH_UNIT(LENGTH_MEASURE(1.E-5),#34877,
'DISTANCE_ACCURACY_VALUE',
'Maximum model space distance between geometric entities at asserted c
onnectivities');
#34841=UNCERTAINTY_MEASURE_WITH_UNIT(LENGTH_MEASURE(1.E-5),#34877,
'DISTANCE_ACCURACY_VALUE',
'Maximum model space distance between geometric entities at asserted c
onnectivities');
#34872=(
GEOMETRIC_REPRESENTATION_CONTEXT(3)
GLOBAL_UNCERTAINTY_ASSIGNED_CONTEXT((#34837))
GLOBAL_UNIT_ASSIGNED_CONTEXT((#34877,#34878,#34879))
REPRESENTATION_CONTEXT('','3D')
);
#34876=(
GEOMETRIC_REPRESENTATION_CONTEXT(3)
GLOBAL_UNCERTAINTY_ASSIGNED_CONTEXT((#34841))
GLOBAL_UNIT_ASSIGNED_CONTEXT((#34877,#34878,#34879))
REPRESENTATION_CONTEXT('','3D')
);
#34877=(
LENGTH_UNIT()
NAMED_UNIT(*)
SI_UNIT($,.METRE.)
);
#34878=(
NAMED_UNIT(*)
PLANE_ANGLE_UNIT()
SI_UNIT($,.RADIAN.)
);
#34879=(
NAMED_UNIT(*)
SI_UNIT($,.STERADIAN.)
SOLID_ANGLE_UNIT()
);
#34910=SHAPE_DEFINITION_REPRESENTATION(#34944,#35014);
#34944=PRODUCT_DEFINITION_SHAPE('',$,#35049);
#35014=SHAPE_REPRESENTATION('',(#22049),#34872);
#35018=PRODUCT_DEFINITION_CONTEXT('part definition',#35122,'design');
#35049=PRODUCT_DEFINITION('Motor Stator Face 8','Motor Stator Face 8',#35083,
#35018);
#35083=PRODUCT_DEFINITION_FORMATION('',$,#35154);
#35122=APPLICATION_CONTEXT('Managed model based 3d engineering');
#35123=PRODUCT_CONTEXT('part definition',#35122,'mechanical');
#35154=PRODUCT('Motor Stator Face 8','Motor Stator Face 8',
'LEGAL AND USAGE DISCLAIMER: this Data/Model is provided \X2\201C\X0\A
S IS\X2\201D\X0\ for informational and representational only. It is a 
geometric approximation and is NOT engineered, certified, or guarantee
d for dimensional accuracy, exact tolerances, or production-level prec
ision. Vendor disclaims all implied warranties including fitness for a
 particular purpose. DO NOT USE FOR DIRECT PHYSICAL MANUFACTURING, AUT
OMATED PRODUCTION, OR SAFETY-CRITICAL SYSTEMS without independent engi
neering verification and resolution of any design discrepancies.',(#35123));
#35163=PRESENTATION_STYLE_ASSIGNMENT((#35172));
#35172=SURFACE_STYLE_USAGE(.BOTH.,#35181);
#35181=SURFACE_SIDE_STYLE('',(#35190));
#35190=SURFACE_STYLE_FILL_AREA(#35199);
#35199=FILL_AREA_STYLE('Plastic - Matte (Black)',(#35208));
#35208=FILL_AREA_STYLE_COLOUR('Plastic - Matte (Black)',#35217);
#35217=COLOUR_RGB('Plastic - Matte (Black)',0.0980392156862745,0.0980392156862745,
0.0980392156862745);
ENDSEC;
END-ISO-10303-21;
